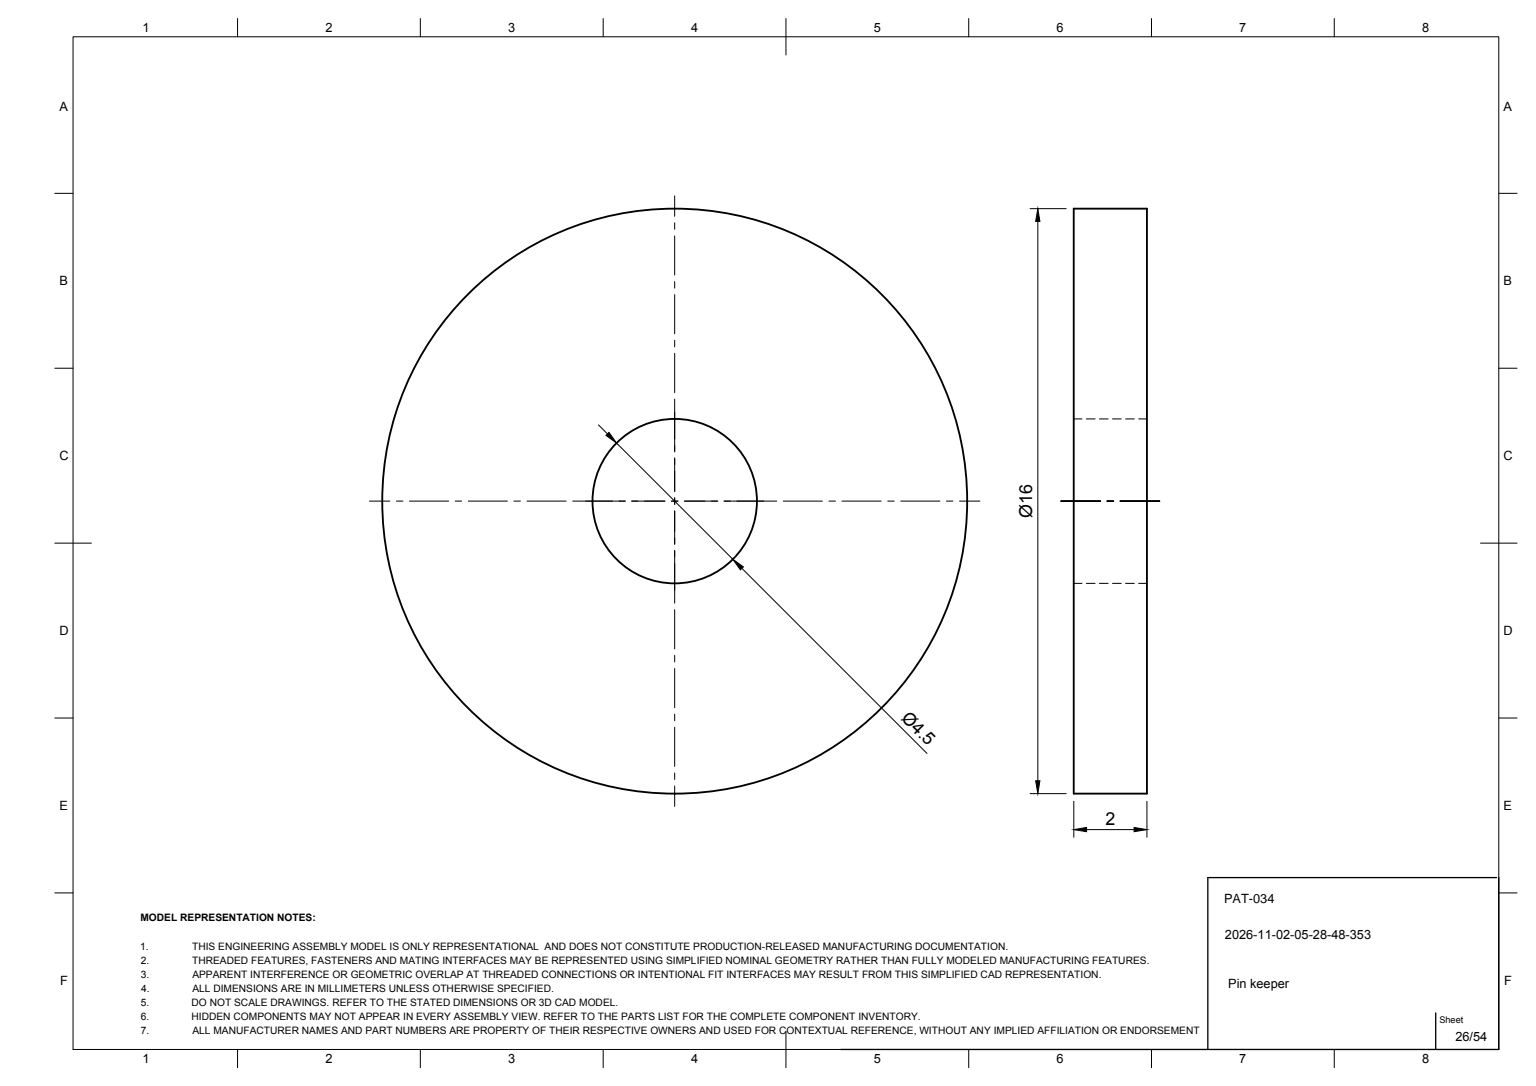
ISO-10303-21;
HEADER;
/* Generated by software containing ST-Developer
 * from STEP Tools, Inc. (www.steptools.com) 
 */

FILE_DESCRIPTION(
/* description */ ('Fatigue rig crank-slider'),
/* implementation_level */ '2;1');

FILE_NAME(
/* name */ 'Pin keeper.step',
/* time_stamp */ '2026-10-28T03:24:50-07:00',
/* author */ (''),
/* organization */ (''),
/* preprocessor_version */ 'ST-DEVELOPER v20.2',
/* originating_system */ 'Autodesk Translation Framework v15.17.0.0',
/* authorisation */ '');

FILE_SCHEMA (('AUTOMOTIVE_DESIGN { 1 0 10303 214 3 1 1 }'));
ENDSEC;

DATA;
#10=MECHANICAL_DESIGN_GEOMETRIC_PRESENTATION_REPRESENTATION('',(#612),#16911);
#511=SHAPE_REPRESENTATION_RELATIONSHIP('SRR','None',#17152,#561);
#561=ADVANCED_BREP_SHAPE_REPRESENTATION('',(#669),#16881);
#612=STYLED_ITEM('',(#17487),#669);
#669=MANIFOLD_SOLID_BREP('Body1',#8905);
#839=FACE_BOUND('',#2157,.T.);
#840=FACE_BOUND('',#2159,.T.);
#1061=PLANE('',#10022);
#1062=PLANE('',#10023);
#1492=FACE_OUTER_BOUND('',#2154,.T.);
#1493=FACE_OUTER_BOUND('',#2155,.T.);
#1494=FACE_OUTER_BOUND('',#2156,.T.);
#1495=FACE_OUTER_BOUND('',#2158,.T.);
#2154=EDGE_LOOP('',(#7146,#7147,#7148,#7149));
#2155=EDGE_LOOP('',(#7150,#7151,#7152,#7153));
#2156=EDGE_LOOP('',(#7154));
#2157=EDGE_LOOP('',(#7155));
#2158=EDGE_LOOP('',(#7156));
#2159=EDGE_LOOP('',(#7157));
#2782=LINE('',#15213,#3428);
#2783=LINE('',#15219,#3429);
#3428=VECTOR('',#11938,0.225);
#3429=VECTOR('',#11945,0.8);
#3969=CIRCLE('',#10017,0.225);
#3970=CIRCLE('',#10018,0.225);
#3971=CIRCLE('',#10020,0.8);
#3972=CIRCLE('',#10021,0.8);
#4541=VERTEX_POINT('',#15210);
#4542=VERTEX_POINT('',#15212);
#4543=VERTEX_POINT('',#15216);
#4544=VERTEX_POINT('',#15218);
#5471=EDGE_CURVE('',#4541,#4541,#3969,.T.);
#5472=EDGE_CURVE('',#4541,#4542,#2782,.T.);
#5473=EDGE_CURVE('',#4542,#4542,#3970,.T.);
#5474=EDGE_CURVE('',#4543,#4543,#3971,.T.);
#5475=EDGE_CURVE('',#4543,#4544,#2783,.T.);
#5476=EDGE_CURVE('',#4544,#4544,#3972,.T.);
#7146=ORIENTED_EDGE('',*,*,#5471,.F.);
#7147=ORIENTED_EDGE('',*,*,#5472,.T.);
#7148=ORIENTED_EDGE('',*,*,#5473,.T.);
#7149=ORIENTED_EDGE('',*,*,#5472,.F.);
#7150=ORIENTED_EDGE('',*,*,#5474,.F.);
#7151=ORIENTED_EDGE('',*,*,#5475,.T.);
#7152=ORIENTED_EDGE('',*,*,#5476,.T.);
#7153=ORIENTED_EDGE('',*,*,#5475,.F.);
#7154=ORIENTED_EDGE('',*,*,#5474,.T.);
#7155=ORIENTED_EDGE('',*,*,#5471,.T.);
#7156=ORIENTED_EDGE('',*,*,#5476,.F.);
#7157=ORIENTED_EDGE('',*,*,#5473,.F.);
#8298=CYLINDRICAL_SURFACE('',#10016,0.225);
#8299=CYLINDRICAL_SURFACE('',#10019,0.8);
#8630=ADVANCED_FACE('',(#1492),#8298,.F.);
#8631=ADVANCED_FACE('',(#1493),#8299,.T.);
#8632=ADVANCED_FACE('',(#1494,#839),#1061,.T.);
#8633=ADVANCED_FACE('',(#1495,#840),#1062,.F.);
#8905=CLOSED_SHELL('',(#8630,#8631,#8632,#8633));
#10015=AXIS2_PLACEMENT_3D('',#15208,#11932,#11933);
#10016=AXIS2_PLACEMENT_3D('',#15209,#11934,#11935);
#10017=AXIS2_PLACEMENT_3D('',#15211,#11936,#11937);
#10018=AXIS2_PLACEMENT_3D('',#15214,#11939,#11940);
#10019=AXIS2_PLACEMENT_3D('',#15215,#11941,#11942);
#10020=AXIS2_PLACEMENT_3D('',#15217,#11943,#11944);
#10021=AXIS2_PLACEMENT_3D('',#15220,#11946,#11947);
#10022=AXIS2_PLACEMENT_3D('',#15221,#11948,#11949);
#10023=AXIS2_PLACEMENT_3D('',#15222,#11950,#11951);
#11932=DIRECTION('axis',(0.,0.,1.));
#11933=DIRECTION('refdir',(1.,0.,0.));
#11934=DIRECTION('center_axis',(0.,1.,0.));
#11935=DIRECTION('ref_axis',(1.,0.,0.));
#11936=DIRECTION('center_axis',(0.,-1.,0.));
#11937=DIRECTION('ref_axis',(1.,0.,0.));
#11938=DIRECTION('',(0.,-1.,0.));
#11939=DIRECTION('center_axis',(0.,-1.,0.));
#11940=DIRECTION('ref_axis',(1.,0.,0.));
#11941=DIRECTION('center_axis',(0.,1.,0.));
#11942=DIRECTION('ref_axis',(1.,0.,0.));
#11943=DIRECTION('center_axis',(0.,1.,0.));
#11944=DIRECTION('ref_axis',(1.,0.,0.));
#11945=DIRECTION('',(0.,-1.,0.));
#11946=DIRECTION('center_axis',(0.,1.,0.));
#11947=DIRECTION('ref_axis',(1.,0.,0.));
#11948=DIRECTION('center_axis',(0.,1.,0.));
#11949=DIRECTION('ref_axis',(1.,0.,0.));
#11950=DIRECTION('center_axis',(0.,1.,0.));
#11951=DIRECTION('ref_axis',(1.,0.,0.));
#15208=CARTESIAN_POINT('',(0.,0.,0.));
#15209=CARTESIAN_POINT('Origin',(1.,4.8,12.));
#15210=CARTESIAN_POINT('',(0.775,5.,12.));
#15211=CARTESIAN_POINT('Origin',(1.,5.,12.));
#15212=CARTESIAN_POINT('',(0.775,4.8,12.));
#15213=CARTESIAN_POINT('',(0.775,4.8,12.));
#15214=CARTESIAN_POINT('Origin',(1.,4.8,12.));
#15215=CARTESIAN_POINT('Origin',(1.,4.8,12.));
#15216=CARTESIAN_POINT('',(0.2,5.,12.));
#15217=CARTESIAN_POINT('Origin',(1.,5.,12.));
#15218=CARTESIAN_POINT('',(0.2,4.8,12.));
#15219=CARTESIAN_POINT('',(0.2,4.8,12.));
#15220=CARTESIAN_POINT('Origin',(1.,4.8,12.));
#15221=CARTESIAN_POINT('Origin',(1.,5.,12.));
#15222=CARTESIAN_POINT('Origin',(1.,4.8,12.));
#16822=UNCERTAINTY_MEASURE_WITH_UNIT(LENGTH_MEASURE(0.001),#16912,
'DISTANCE_ACCURACY_VALUE',
'Maximum model space distance between geometric entities at asserted c
onnectivities');
#16852=UNCERTAINTY_MEASURE_WITH_UNIT(LENGTH_MEASURE(0.001),#16912,
'DISTANCE_ACCURACY_VALUE',
'Maximum model space distance between geometric entities at asserted c
onnectivities');
#16881=(
GEOMETRIC_REPRESENTATION_CONTEXT(3)
GLOBAL_UNCERTAINTY_ASSIGNED_CONTEXT((#16822))
GLOBAL_UNIT_ASSIGNED_CONTEXT((#16912,#16914,#16915))
REPRESENTATION_CONTEXT('','3D')
);
#16911=(
GEOMETRIC_REPRESENTATION_CONTEXT(3)
GLOBAL_UNCERTAINTY_ASSIGNED_CONTEXT((#16852))
GLOBAL_UNIT_ASSIGNED_CONTEXT((#16912,#16914,#16915))
REPRESENTATION_CONTEXT('','3D')
);
#16912=(
LENGTH_UNIT()
NAMED_UNIT(*)
SI_UNIT(.CENTI.,.METRE.)
);
#16914=(
NAMED_UNIT(*)
PLANE_ANGLE_UNIT()
SI_UNIT($,.RADIAN.)
);
#16915=(
NAMED_UNIT(*)
SI_UNIT($,.STERADIAN.)
SOLID_ANGLE_UNIT()
);
#16944=SHAPE_DEFINITION_REPRESENTATION(#17004,#17152);
#17004=PRODUCT_DEFINITION_SHAPE('',$,#17211);
#17152=SHAPE_REPRESENTATION('',(#10015),#16881);
#17182=PRODUCT_DEFINITION_CONTEXT('part definition',#17358,'design');
#17211=PRODUCT_DEFINITION('Pin keeper','Pin keeper',#17269,#17182);
#17269=PRODUCT_DEFINITION_FORMATION('',$,#17388);
#17358=APPLICATION_CONTEXT(
'Core Data for Automotive Mechanical Design Process');
#17359=PRODUCT_CONTEXT('part definition',#17358,'mechanical');
#17388=PRODUCT('Pin keeper','Pin keeper','Pin keeper',(#17359));
#17481=COLOUR_RGB('Grey',0.48,0.52,0.57);
#17482=FILL_AREA_STYLE_COLOUR('',#17481);
#17483=FILL_AREA_STYLE('',(#17482));
#17484=SURFACE_STYLE_FILL_AREA(#17483);
#17485=SURFACE_SIDE_STYLE('',(#17484));
#17486=SURFACE_STYLE_USAGE(.BOTH.,#17485);
#17487=PRESENTATION_STYLE_ASSIGNMENT((#17486));
ENDSEC;
END-ISO-10303-21;
